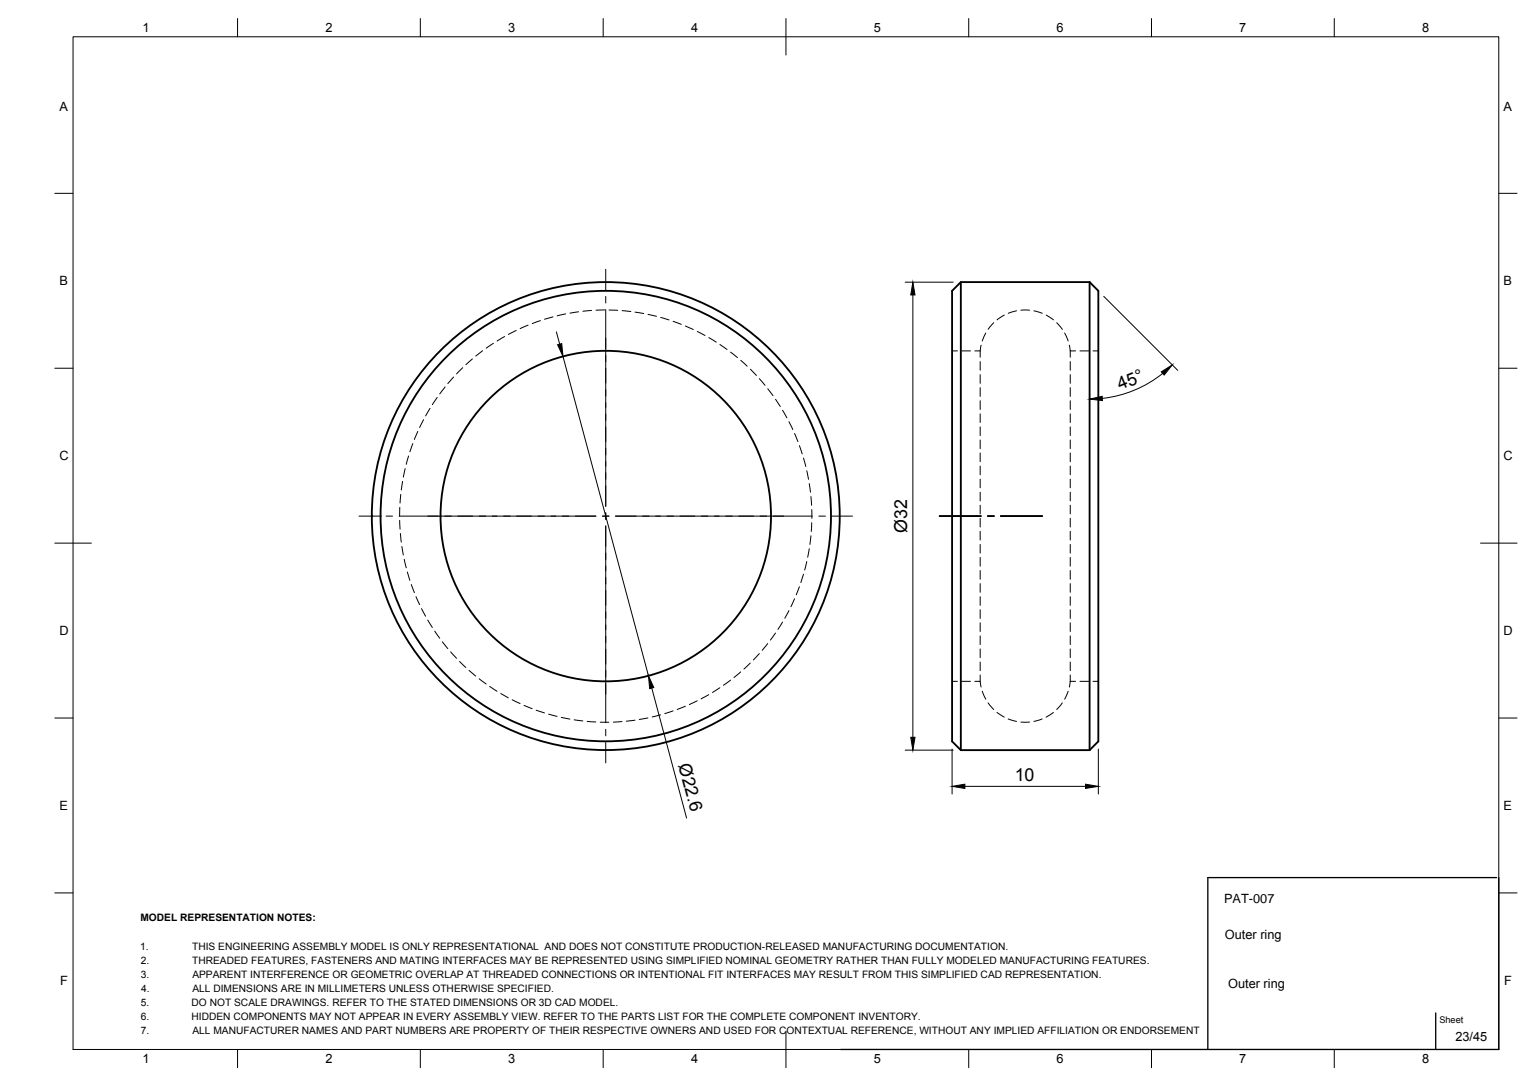
ISO-10303-21;
HEADER;
/* Generated by software containing ST-Developer
 * from STEP Tools, Inc. (www.steptools.com) 
 */

FILE_DESCRIPTION(
/* description */ ('Bearing friction torque test rig'),
/* implementation_level */ '2;1');

FILE_NAME(
/* name */ 'Outer ring.step',
/* time_stamp */ '2026-10-28T03:24:04-07:00',
/* author */ (''),
/* organization */ (''),
/* preprocessor_version */ 'ST-DEVELOPER v20.2',
/* originating_system */ 'Autodesk Translation Framework v15.17.0.0',
/* authorisation */ '');

FILE_SCHEMA (('AUTOMOTIVE_DESIGN { 1 0 10303 214 3 1 1 }'));
ENDSEC;

DATA;
#10=MECHANICAL_DESIGN_GEOMETRIC_PRESENTATION_REPRESENTATION('',(#556),#14822);
#426=TOROIDAL_SURFACE('',#8644,1.1,0.309556);
#434=CONICAL_SURFACE('',#8655,1.57,0.785398163397449);
#435=CONICAL_SURFACE('',#8659,1.57,0.785398163397449);
#478=SHAPE_REPRESENTATION_RELATIONSHIP('SRR','None',#15018,#517);
#517=ADVANCED_BREP_SHAPE_REPRESENTATION('',(#609),#14798);
#556=STYLED_ITEM('',(#15284),#609);
#609=MANIFOLD_SOLID_BREP('Body1',#7673);
#816=FACE_BOUND('',#1964,.T.);
#817=FACE_BOUND('',#1969,.T.);
#1004=PLANE('',#8652);
#1005=PLANE('',#8661);
#1344=FACE_OUTER_BOUND('',#1961,.T.);
#1345=FACE_OUTER_BOUND('',#1962,.T.);
#1346=FACE_OUTER_BOUND('',#1963,.T.);
#1347=FACE_OUTER_BOUND('',#1965,.T.);
#1348=FACE_OUTER_BOUND('',#1966,.T.);
#1349=FACE_OUTER_BOUND('',#1967,.T.);
#1350=FACE_OUTER_BOUND('',#1968,.T.);
#1351=FACE_OUTER_BOUND('',#1970,.T.);
#1961=EDGE_LOOP('',(#6236,#6237,#6238,#6239,#6240,#6241));
#1962=EDGE_LOOP('',(#6242,#6243,#6244,#6245,#6246));
#1963=EDGE_LOOP('',(#6247));
#1964=EDGE_LOOP('',(#6248));
#1965=EDGE_LOOP('',(#6249,#6250,#6251,#6252));
#1966=EDGE_LOOP('',(#6253,#6254,#6255,#6256));
#1967=EDGE_LOOP('',(#6257,#6258,#6259,#6260));
#1968=EDGE_LOOP('',(#6261));
#1969=EDGE_LOOP('',(#6262));
#1970=EDGE_LOOP('',(#6263,#6264,#6265,#6266,#6267));
#2527=LINE('',#12842,#2971);
#2528=LINE('',#12851,#2972);
#2529=LINE('',#12855,#2973);
#2530=LINE('',#12859,#2974);
#2531=LINE('',#12862,#2975);
#2971=VECTOR('',#10494,1.129765);
#2972=VECTOR('',#10505,1.57);
#2973=VECTOR('',#10510,1.6);
#2974=VECTOR('',#10515,1.57);
#2975=VECTOR('',#10520,1.129765);
#3337=CIRCLE('',#8645,1.129765);
#3338=CIRCLE('',#8646,1.129765);
#3339=CIRCLE('',#8647,0.309556);
#3340=CIRCLE('',#8648,1.129765);
#3341=CIRCLE('',#8649,1.129765);
#3342=CIRCLE('',#8651,1.129765);
#3343=CIRCLE('',#8653,1.54);
#3344=CIRCLE('',#8654,1.129765);
#3345=CIRCLE('',#8656,1.6);
#3346=CIRCLE('',#8658,1.6);
#3347=CIRCLE('',#8660,1.54);
#3914=VERTEX_POINT('',#12830);
#3915=VERTEX_POINT('',#12831);
#3916=VERTEX_POINT('',#12834);
#3917=VERTEX_POINT('',#12836);
#3918=VERTEX_POINT('',#12840);
#3919=VERTEX_POINT('',#12844);
#3920=VERTEX_POINT('',#12846);
#3921=VERTEX_POINT('',#12849);
#3922=VERTEX_POINT('',#12853);
#3923=VERTEX_POINT('',#12857);
#4744=EDGE_CURVE('',#3914,#3915,#3337,.T.);
#4745=EDGE_CURVE('',#3915,#3914,#3338,.T.);
#4746=EDGE_CURVE('',#3915,#3916,#3339,.T.);
#4747=EDGE_CURVE('',#3917,#3916,#3340,.T.);
#4748=EDGE_CURVE('',#3916,#3917,#3341,.T.);
#4749=EDGE_CURVE('',#3918,#3918,#3342,.T.);
#4750=EDGE_CURVE('',#3918,#3917,#2527,.T.);
#4751=EDGE_CURVE('',#3919,#3919,#3343,.T.);
#4752=EDGE_CURVE('',#3920,#3920,#3344,.T.);
#4753=EDGE_CURVE('',#3921,#3921,#3345,.T.);
#4754=EDGE_CURVE('',#3921,#3919,#2528,.T.);
#4755=EDGE_CURVE('',#3922,#3922,#3346,.T.);
#4756=EDGE_CURVE('',#3922,#3921,#2529,.T.);
#4757=EDGE_CURVE('',#3923,#3923,#3347,.T.);
#4758=EDGE_CURVE('',#3923,#3922,#2530,.T.);
#4759=EDGE_CURVE('',#3914,#3920,#2531,.T.);
#6236=ORIENTED_EDGE('',*,*,#4744,.F.);
#6237=ORIENTED_EDGE('',*,*,#4745,.F.);
#6238=ORIENTED_EDGE('',*,*,#4746,.T.);
#6239=ORIENTED_EDGE('',*,*,#4747,.F.);
#6240=ORIENTED_EDGE('',*,*,#4748,.F.);
#6241=ORIENTED_EDGE('',*,*,#4746,.F.);
#6242=ORIENTED_EDGE('',*,*,#4749,.T.);
#6243=ORIENTED_EDGE('',*,*,#4750,.T.);
#6244=ORIENTED_EDGE('',*,*,#4747,.T.);
#6245=ORIENTED_EDGE('',*,*,#4748,.T.);
#6246=ORIENTED_EDGE('',*,*,#4750,.F.);
#6247=ORIENTED_EDGE('',*,*,#4751,.F.);
#6248=ORIENTED_EDGE('',*,*,#4752,.T.);
#6249=ORIENTED_EDGE('',*,*,#4753,.F.);
#6250=ORIENTED_EDGE('',*,*,#4754,.T.);
#6251=ORIENTED_EDGE('',*,*,#4751,.T.);
#6252=ORIENTED_EDGE('',*,*,#4754,.F.);
#6253=ORIENTED_EDGE('',*,*,#4755,.F.);
#6254=ORIENTED_EDGE('',*,*,#4756,.T.);
#6255=ORIENTED_EDGE('',*,*,#4753,.T.);
#6256=ORIENTED_EDGE('',*,*,#4756,.F.);
#6257=ORIENTED_EDGE('',*,*,#4757,.F.);
#6258=ORIENTED_EDGE('',*,*,#4758,.T.);
#6259=ORIENTED_EDGE('',*,*,#4755,.T.);
#6260=ORIENTED_EDGE('',*,*,#4758,.F.);
#6261=ORIENTED_EDGE('',*,*,#4757,.T.);
#6262=ORIENTED_EDGE('',*,*,#4749,.F.);
#6263=ORIENTED_EDGE('',*,*,#4744,.T.);
#6264=ORIENTED_EDGE('',*,*,#4745,.T.);
#6265=ORIENTED_EDGE('',*,*,#4759,.T.);
#6266=ORIENTED_EDGE('',*,*,#4752,.F.);
#6267=ORIENTED_EDGE('',*,*,#4759,.F.);
#7153=CYLINDRICAL_SURFACE('',#8650,1.129765);
#7154=CYLINDRICAL_SURFACE('',#8657,1.6);
#7155=CYLINDRICAL_SURFACE('',#8662,1.129765);
#7455=ADVANCED_FACE('',(#1344),#426,.F.);
#7456=ADVANCED_FACE('',(#1345),#7153,.F.);
#7457=ADVANCED_FACE('',(#1346,#816),#1004,.T.);
#7458=ADVANCED_FACE('',(#1347),#434,.T.);
#7459=ADVANCED_FACE('',(#1348),#7154,.T.);
#7460=ADVANCED_FACE('',(#1349),#435,.T.);
#7461=ADVANCED_FACE('',(#1350,#817),#1005,.T.);
#7462=ADVANCED_FACE('',(#1351),#7155,.F.);
#7673=CLOSED_SHELL('',(#7455,#7456,#7457,#7458,#7459,#7460,#7461,#7462));
#8643=AXIS2_PLACEMENT_3D('',#12828,#10476,#10477);
#8644=AXIS2_PLACEMENT_3D('',#12829,#10478,#10479);
#8645=AXIS2_PLACEMENT_3D('',#12832,#10480,#10481);
#8646=AXIS2_PLACEMENT_3D('',#12833,#10482,#10483);
#8647=AXIS2_PLACEMENT_3D('',#12835,#10484,#10485);
#8648=AXIS2_PLACEMENT_3D('',#12837,#10486,#10487);
#8649=AXIS2_PLACEMENT_3D('',#12838,#10488,#10489);
#8650=AXIS2_PLACEMENT_3D('',#12839,#10490,#10491);
#8651=AXIS2_PLACEMENT_3D('',#12841,#10492,#10493);
#8652=AXIS2_PLACEMENT_3D('',#12843,#10495,#10496);
#8653=AXIS2_PLACEMENT_3D('',#12845,#10497,#10498);
#8654=AXIS2_PLACEMENT_3D('',#12847,#10499,#10500);
#8655=AXIS2_PLACEMENT_3D('',#12848,#10501,#10502);
#8656=AXIS2_PLACEMENT_3D('',#12850,#10503,#10504);
#8657=AXIS2_PLACEMENT_3D('',#12852,#10506,#10507);
#8658=AXIS2_PLACEMENT_3D('',#12854,#10508,#10509);
#8659=AXIS2_PLACEMENT_3D('',#12856,#10511,#10512);
#8660=AXIS2_PLACEMENT_3D('',#12858,#10513,#10514);
#8661=AXIS2_PLACEMENT_3D('',#12860,#10516,#10517);
#8662=AXIS2_PLACEMENT_3D('',#12861,#10518,#10519);
#10476=DIRECTION('axis',(0.,0.,1.));
#10477=DIRECTION('refdir',(1.,0.,0.));
#10478=DIRECTION('center_axis',(0.,-1.,0.));
#10479=DIRECTION('ref_axis',(0.,0.,-1.));
#10480=DIRECTION('center_axis',(0.,-1.,0.));
#10481=DIRECTION('ref_axis',(1.,0.,0.));
#10482=DIRECTION('center_axis',(0.,-1.,0.));
#10483=DIRECTION('ref_axis',(1.,0.,0.));
#10484=DIRECTION('center_axis',(1.,0.,1.22464679914735E-16));
#10485=DIRECTION('ref_axis',(-1.22464679914735E-16,0.,1.));
#10486=DIRECTION('center_axis',(0.,1.,0.));
#10487=DIRECTION('ref_axis',(1.,0.,0.));
#10488=DIRECTION('center_axis',(0.,1.,0.));
#10489=DIRECTION('ref_axis',(1.,0.,0.));
#10490=DIRECTION('center_axis',(0.,-1.,0.));
#10491=DIRECTION('ref_axis',(1.,0.,0.));
#10492=DIRECTION('center_axis',(0.,-1.,0.));
#10493=DIRECTION('ref_axis',(1.,0.,0.));
#10494=DIRECTION('',(0.,1.,0.));
#10495=DIRECTION('center_axis',(0.,1.,0.));
#10496=DIRECTION('ref_axis',(0.,0.,1.));
#10497=DIRECTION('center_axis',(0.,-1.,0.));
#10498=DIRECTION('ref_axis',(1.,0.,0.));
#10499=DIRECTION('center_axis',(0.,-1.,0.));
#10500=DIRECTION('ref_axis',(1.,0.,0.));
#10501=DIRECTION('center_axis',(0.,-1.,0.));
#10502=DIRECTION('ref_axis',(1.,0.,0.));
#10503=DIRECTION('center_axis',(0.,-1.,0.));
#10504=DIRECTION('ref_axis',(1.,0.,0.));
#10505=DIRECTION('',(0.707106781186548,0.707106781186547,8.65956056235494E-17));
#10506=DIRECTION('center_axis',(0.,-1.,0.));
#10507=DIRECTION('ref_axis',(1.,0.,0.));
#10508=DIRECTION('center_axis',(0.,-1.,0.));
#10509=DIRECTION('ref_axis',(1.,0.,0.));
#10510=DIRECTION('',(0.,1.,0.));
#10511=DIRECTION('center_axis',(0.,1.,0.));
#10512=DIRECTION('ref_axis',(1.,0.,0.));
#10513=DIRECTION('center_axis',(0.,-1.,0.));
#10514=DIRECTION('ref_axis',(1.,0.,0.));
#10515=DIRECTION('',(-0.707106781186548,0.707106781186547,-8.65956056235494E-17));
#10516=DIRECTION('center_axis',(0.,-1.,0.));
#10517=DIRECTION('ref_axis',(0.,0.,-1.));
#10518=DIRECTION('center_axis',(0.,-1.,0.));
#10519=DIRECTION('ref_axis',(1.,0.,0.));
#10520=DIRECTION('',(0.,1.,0.));
#12828=CARTESIAN_POINT('',(0.,0.,0.));
#12829=CARTESIAN_POINT('Origin',(0.,0.,0.));
#12830=CARTESIAN_POINT('',(-1.129765,0.308121667383195,-1.38356309103871E-16));
#12831=CARTESIAN_POINT('',(-1.38356309103871E-16,0.308121667383195,1.129765));
#12832=CARTESIAN_POINT('Origin',(0.,0.308121667383195,0.));
#12833=CARTESIAN_POINT('Origin',(0.,0.308121667383195,0.));
#12834=CARTESIAN_POINT('',(-1.38356309103871E-16,-0.308121667383195,1.129765));
#12835=CARTESIAN_POINT('Origin',(-1.34711147906209E-16,0.,1.1));
#12836=CARTESIAN_POINT('',(-1.129765,-0.308121667383195,1.38356309103871E-16));
#12837=CARTESIAN_POINT('Origin',(0.,-0.308121667383195,0.));
#12838=CARTESIAN_POINT('Origin',(0.,-0.308121667383195,0.));
#12839=CARTESIAN_POINT('Origin',(0.,0.,0.));
#12840=CARTESIAN_POINT('',(-1.129765,-0.5,-1.38356309103871E-16));
#12841=CARTESIAN_POINT('Origin',(0.,-0.5,0.));
#12842=CARTESIAN_POINT('',(-1.129765,0.,-1.38356309103871E-16));
#12843=CARTESIAN_POINT('Origin',(1.54,0.5,0.));
#12844=CARTESIAN_POINT('',(-1.54,0.5,-1.88595607068692E-16));
#12845=CARTESIAN_POINT('Origin',(0.,0.5,0.));
#12846=CARTESIAN_POINT('',(-1.129765,0.5,-1.38356309103871E-16));
#12847=CARTESIAN_POINT('Origin',(0.,0.5,0.));
#12848=CARTESIAN_POINT('Origin',(0.,0.47,0.));
#12849=CARTESIAN_POINT('',(-1.6,0.44,-1.95943487863577E-16));
#12850=CARTESIAN_POINT('Origin',(0.,0.44,0.));
#12851=CARTESIAN_POINT('',(-1.57,0.47,-1.92269547466134E-16));
#12852=CARTESIAN_POINT('Origin',(0.,0.,0.));
#12853=CARTESIAN_POINT('',(-1.6,-0.44,-1.95943487863577E-16));
#12854=CARTESIAN_POINT('Origin',(0.,-0.44,0.));
#12855=CARTESIAN_POINT('',(-1.6,0.,-1.95943487863577E-16));
#12856=CARTESIAN_POINT('Origin',(0.,-0.47,0.));
#12857=CARTESIAN_POINT('',(-1.54,-0.5,-1.88595607068692E-16));
#12858=CARTESIAN_POINT('Origin',(0.,-0.5,0.));
#12859=CARTESIAN_POINT('',(-1.57,-0.47,-1.92269547466134E-16));
#12860=CARTESIAN_POINT('Origin',(1.129765,-0.5,0.));
#12861=CARTESIAN_POINT('Origin',(0.,0.,0.));
#12862=CARTESIAN_POINT('',(-1.129765,0.,-1.38356309103871E-16));
#14753=UNCERTAINTY_MEASURE_WITH_UNIT(LENGTH_MEASURE(0.001),#14823,
'DISTANCE_ACCURACY_VALUE',
'Maximum model space distance between geometric entities at asserted c
onnectivities');
#14777=UNCERTAINTY_MEASURE_WITH_UNIT(LENGTH_MEASURE(0.001),#14823,
'DISTANCE_ACCURACY_VALUE',
'Maximum model space distance between geometric entities at asserted c
onnectivities');
#14798=(
GEOMETRIC_REPRESENTATION_CONTEXT(3)
GLOBAL_UNCERTAINTY_ASSIGNED_CONTEXT((#14753))
GLOBAL_UNIT_ASSIGNED_CONTEXT((#14823,#14825,#14826))
REPRESENTATION_CONTEXT('','3D')
);
#14822=(
GEOMETRIC_REPRESENTATION_CONTEXT(3)
GLOBAL_UNCERTAINTY_ASSIGNED_CONTEXT((#14777))
GLOBAL_UNIT_ASSIGNED_CONTEXT((#14823,#14825,#14826))
REPRESENTATION_CONTEXT('','3D')
);
#14823=(
LENGTH_UNIT()
NAMED_UNIT(*)
SI_UNIT(.CENTI.,.METRE.)
);
#14825=(
NAMED_UNIT(*)
PLANE_ANGLE_UNIT()
SI_UNIT($,.RADIAN.)
);
#14826=(
NAMED_UNIT(*)
SI_UNIT($,.STERADIAN.)
SOLID_ANGLE_UNIT()
);
#14847=SHAPE_DEFINITION_REPRESENTATION(#14891,#15018);
#14891=PRODUCT_DEFINITION_SHAPE('',$,#15063);
#15018=SHAPE_REPRESENTATION('',(#8643),#14798);
#15042=PRODUCT_DEFINITION_CONTEXT('part definition',#15176,'design');
#15063=PRODUCT_DEFINITION('Outer ring','Outer ring',#15107,#15042);
#15107=PRODUCT_DEFINITION_FORMATION('',$,#15198);
#15176=APPLICATION_CONTEXT(
'Core Data for Automotive Mechanical Design Process');
#15177=PRODUCT_CONTEXT('part definition',#15176,'mechanical');
#15198=PRODUCT('Outer ring','Outer ring','Outer ring',(#15177));
#15278=COLOUR_RGB('Grey',0.48,0.52,0.57);
#15279=FILL_AREA_STYLE_COLOUR('',#15278);
#15280=FILL_AREA_STYLE('',(#15279));
#15281=SURFACE_STYLE_FILL_AREA(#15280);
#15282=SURFACE_SIDE_STYLE('',(#15281));
#15283=SURFACE_STYLE_USAGE(.BOTH.,#15282);
#15284=PRESENTATION_STYLE_ASSIGNMENT((#15283));
ENDSEC;
END-ISO-10303-21;
